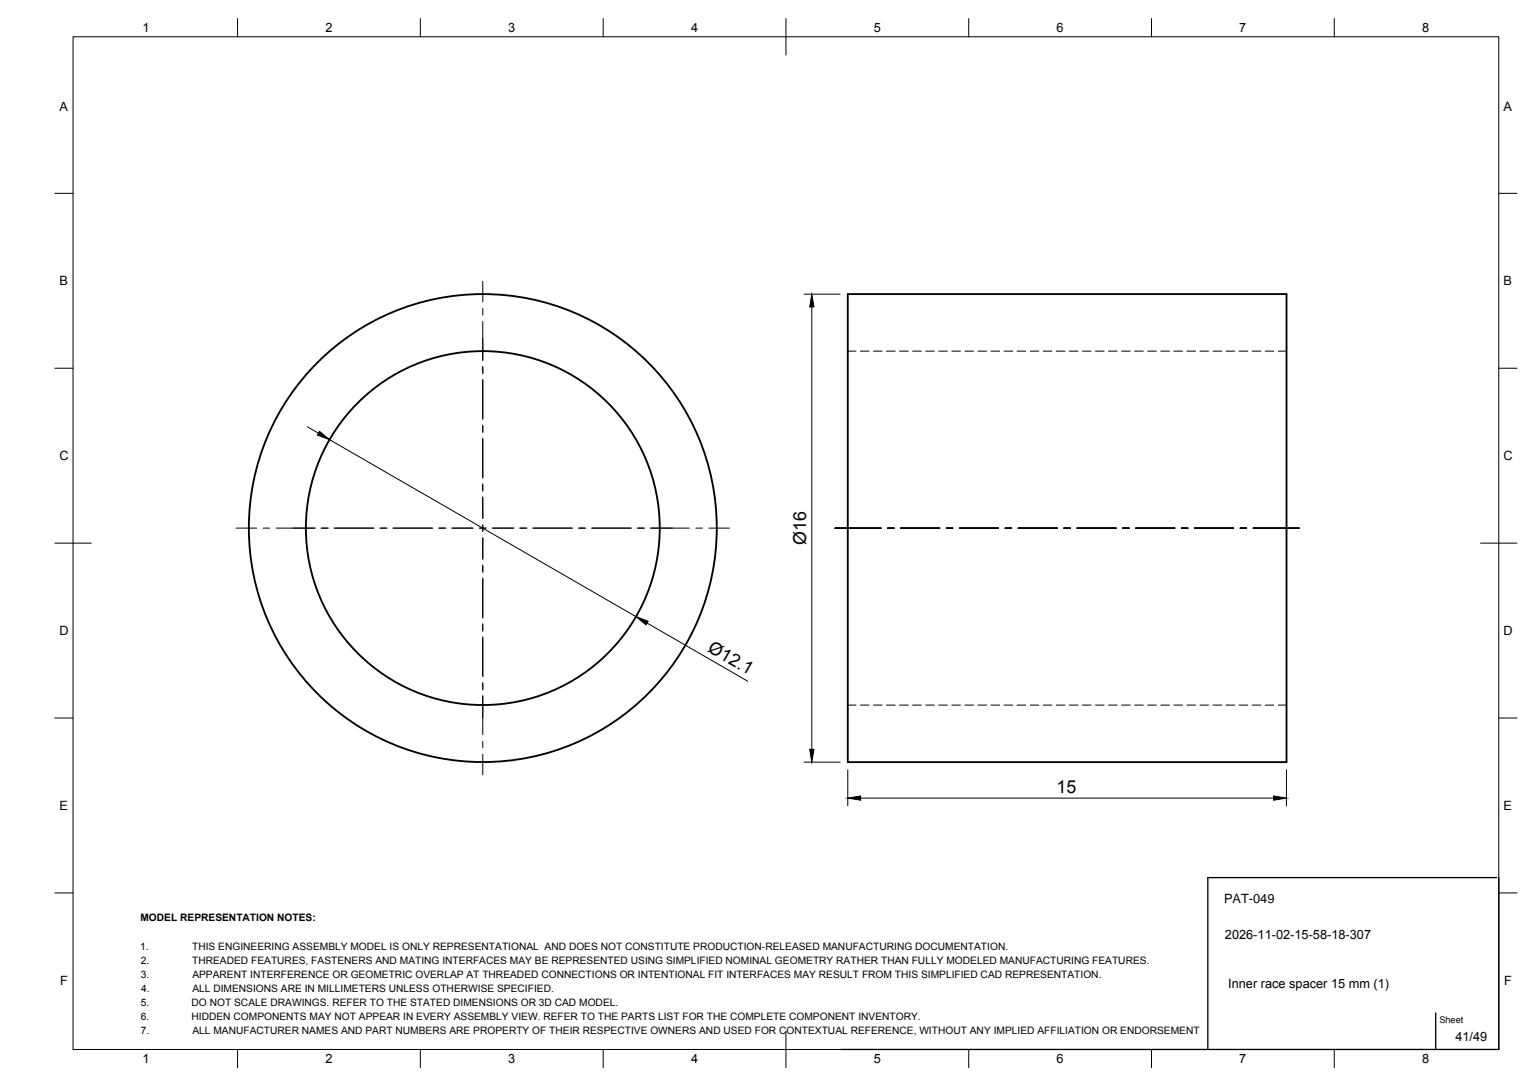
ISO-10303-21;
HEADER;
/* Generated by software containing ST-Developer
 * from STEP Tools, Inc. (www.steptools.com) 
 */

FILE_DESCRIPTION(
/* description */ ('Hand drill press frame (manual)'),
/* implementation_level */ '2;1');

FILE_NAME(
/* name */ 'Inner race spacer 15 mm (1).step',
/* time_stamp */ '2026-10-28T03:25:28-07:00',
/* author */ (''),
/* organization */ (''),
/* preprocessor_version */ 'ST-DEVELOPER v20.2',
/* originating_system */ 'Autodesk Translation Framework v15.17.0.0',
/* authorisation */ '');

FILE_SCHEMA (('AUTOMOTIVE_DESIGN { 1 0 10303 214 3 1 1 }'));
ENDSEC;

DATA;
#10=MECHANICAL_DESIGN_GEOMETRIC_PRESENTATION_REPRESENTATION('',(#659),#33299);
#562=SHAPE_REPRESENTATION_RELATIONSHIP('SRR','None',#33524,#607);
#607=ADVANCED_BREP_SHAPE_REPRESENTATION('',(#710),#33286);
#659=STYLED_ITEM('',(#33814),#710);
#710=MANIFOLD_SOLID_BREP('Body1',#12678);
#865=FACE_BOUND('',#2694,.T.);
#866=FACE_BOUND('',#2696,.T.);
#1258=PLANE('',#14067);
#1259=PLANE('',#14068);
#1857=FACE_OUTER_BOUND('',#2691,.T.);
#1858=FACE_OUTER_BOUND('',#2692,.T.);
#1859=FACE_OUTER_BOUND('',#2693,.T.);
#1860=FACE_OUTER_BOUND('',#2695,.T.);
#2691=EDGE_LOOP('',(#10967,#10968,#10969,#10970));
#2692=EDGE_LOOP('',(#10971,#10972,#10973,#10974));
#2693=EDGE_LOOP('',(#10975));
#2694=EDGE_LOOP('',(#10976));
#2695=EDGE_LOOP('',(#10977));
#2696=EDGE_LOOP('',(#10978));
#3814=LINE('',#21189,#4979);
#3815=LINE('',#21195,#4980);
#4979=VECTOR('',#17047,0.605);
#4980=VECTOR('',#17054,0.8);
#5519=CIRCLE('',#14062,0.605);
#5520=CIRCLE('',#14063,0.605);
#5521=CIRCLE('',#14065,0.8);
#5522=CIRCLE('',#14066,0.8);
#6469=VERTEX_POINT('',#21186);
#6470=VERTEX_POINT('',#21188);
#6471=VERTEX_POINT('',#21192);
#6472=VERTEX_POINT('',#21194);
#8012=EDGE_CURVE('',#6469,#6469,#5519,.T.);
#8013=EDGE_CURVE('',#6469,#6470,#3814,.T.);
#8014=EDGE_CURVE('',#6470,#6470,#5520,.T.);
#8015=EDGE_CURVE('',#6471,#6471,#5521,.T.);
#8016=EDGE_CURVE('',#6471,#6472,#3815,.T.);
#8017=EDGE_CURVE('',#6472,#6472,#5522,.T.);
#10967=ORIENTED_EDGE('',*,*,#8012,.F.);
#10968=ORIENTED_EDGE('',*,*,#8013,.T.);
#10969=ORIENTED_EDGE('',*,*,#8014,.T.);
#10970=ORIENTED_EDGE('',*,*,#8013,.F.);
#10971=ORIENTED_EDGE('',*,*,#8015,.F.);
#10972=ORIENTED_EDGE('',*,*,#8016,.T.);
#10973=ORIENTED_EDGE('',*,*,#8017,.T.);
#10974=ORIENTED_EDGE('',*,*,#8016,.F.);
#10975=ORIENTED_EDGE('',*,*,#8015,.T.);
#10976=ORIENTED_EDGE('',*,*,#8012,.T.);
#10977=ORIENTED_EDGE('',*,*,#8017,.F.);
#10978=ORIENTED_EDGE('',*,*,#8014,.F.);
#11906=CYLINDRICAL_SURFACE('',#14061,0.605);
#11907=CYLINDRICAL_SURFACE('',#14064,0.8);
#12466=ADVANCED_FACE('',(#1857),#11906,.F.);
#12467=ADVANCED_FACE('',(#1858),#11907,.T.);
#12468=ADVANCED_FACE('',(#1859,#865),#1258,.T.);
#12469=ADVANCED_FACE('',(#1860,#866),#1259,.F.);
#12678=CLOSED_SHELL('',(#12466,#12467,#12468,#12469));
#14060=AXIS2_PLACEMENT_3D('',#21184,#17041,#17042);
#14061=AXIS2_PLACEMENT_3D('',#21185,#17043,#17044);
#14062=AXIS2_PLACEMENT_3D('',#21187,#17045,#17046);
#14063=AXIS2_PLACEMENT_3D('',#21190,#17048,#17049);
#14064=AXIS2_PLACEMENT_3D('',#21191,#17050,#17051);
#14065=AXIS2_PLACEMENT_3D('',#21193,#17052,#17053);
#14066=AXIS2_PLACEMENT_3D('',#21196,#17055,#17056);
#14067=AXIS2_PLACEMENT_3D('',#21197,#17057,#17058);
#14068=AXIS2_PLACEMENT_3D('',#21198,#17059,#17060);
#17041=DIRECTION('axis',(0.,0.,1.));
#17042=DIRECTION('refdir',(1.,0.,0.));
#17043=DIRECTION('center_axis',(0.,1.,0.));
#17044=DIRECTION('ref_axis',(1.,0.,0.));
#17045=DIRECTION('center_axis',(0.,-1.,0.));
#17046=DIRECTION('ref_axis',(1.,0.,0.));
#17047=DIRECTION('',(0.,-1.,0.));
#17048=DIRECTION('center_axis',(0.,-1.,0.));
#17049=DIRECTION('ref_axis',(1.,0.,0.));
#17050=DIRECTION('center_axis',(0.,1.,0.));
#17051=DIRECTION('ref_axis',(1.,0.,0.));
#17052=DIRECTION('center_axis',(0.,1.,0.));
#17053=DIRECTION('ref_axis',(1.,0.,0.));
#17054=DIRECTION('',(0.,-1.,0.));
#17055=DIRECTION('center_axis',(0.,1.,0.));
#17056=DIRECTION('ref_axis',(1.,0.,0.));
#17057=DIRECTION('center_axis',(0.,1.,0.));
#17058=DIRECTION('ref_axis',(1.,0.,0.));
#17059=DIRECTION('center_axis',(0.,1.,0.));
#17060=DIRECTION('ref_axis',(1.,0.,0.));
#21184=CARTESIAN_POINT('',(0.,0.,0.));
#21185=CARTESIAN_POINT('Origin',(-3.25,3.5,20.));
#21186=CARTESIAN_POINT('',(-3.855,5.,20.));
#21187=CARTESIAN_POINT('Origin',(-3.25,5.,20.));
#21188=CARTESIAN_POINT('',(-3.855,3.5,20.));
#21189=CARTESIAN_POINT('',(-3.855,3.5,20.));
#21190=CARTESIAN_POINT('Origin',(-3.25,3.5,20.));
#21191=CARTESIAN_POINT('Origin',(-3.25,3.5,20.));
#21192=CARTESIAN_POINT('',(-4.05,5.,20.));
#21193=CARTESIAN_POINT('Origin',(-3.25,5.,20.));
#21194=CARTESIAN_POINT('',(-4.05,3.5,20.));
#21195=CARTESIAN_POINT('',(-4.05,3.5,20.));
#21196=CARTESIAN_POINT('Origin',(-3.25,3.5,20.));
#21197=CARTESIAN_POINT('Origin',(-3.25,5.,20.));
#21198=CARTESIAN_POINT('Origin',(-3.25,3.5,20.));
#33234=UNCERTAINTY_MEASURE_WITH_UNIT(LENGTH_MEASURE(0.001),#33300,
'DISTANCE_ACCURACY_VALUE',
'Maximum model space distance between geometric entities at asserted c
onnectivities');
#33247=UNCERTAINTY_MEASURE_WITH_UNIT(LENGTH_MEASURE(0.001),#33300,
'DISTANCE_ACCURACY_VALUE',
'Maximum model space distance between geometric entities at asserted c
onnectivities');
#33286=(
GEOMETRIC_REPRESENTATION_CONTEXT(3)
GLOBAL_UNCERTAINTY_ASSIGNED_CONTEXT((#33234))
GLOBAL_UNIT_ASSIGNED_CONTEXT((#33300,#33302,#33303))
REPRESENTATION_CONTEXT('','3D')
);
#33299=(
GEOMETRIC_REPRESENTATION_CONTEXT(3)
GLOBAL_UNCERTAINTY_ASSIGNED_CONTEXT((#33247))
GLOBAL_UNIT_ASSIGNED_CONTEXT((#33300,#33302,#33303))
REPRESENTATION_CONTEXT('','3D')
);
#33300=(
LENGTH_UNIT()
NAMED_UNIT(*)
SI_UNIT(.CENTI.,.METRE.)
);
#33302=(
NAMED_UNIT(*)
PLANE_ANGLE_UNIT()
SI_UNIT($,.RADIAN.)
);
#33303=(
NAMED_UNIT(*)
SI_UNIT($,.STERADIAN.)
SOLID_ANGLE_UNIT()
);
#33342=SHAPE_DEFINITION_REPRESENTATION(#33404,#33524);
#33404=PRODUCT_DEFINITION_SHAPE('',$,#33576);
#33524=SHAPE_REPRESENTATION('',(#14060),#33286);
#33537=PRODUCT_DEFINITION_CONTEXT('part definition',#33692,'design');
#33576=PRODUCT_DEFINITION('Inner race spacer 15 mm (1)',
'Inner race spacer 15 mm (1)',#33627,#33537);
#33627=PRODUCT_DEFINITION_FORMATION('',$,#33732);
#33692=APPLICATION_CONTEXT(
'Core Data for Automotive Mechanical Design Process');
#33693=PRODUCT_CONTEXT('part definition',#33692,'mechanical');
#33732=PRODUCT('Inner race spacer 15 mm (1)',
'Inner race spacer 15 mm (1)','Inner race spacer 15 mm (1)',(#33693));
#33808=COLOUR_RGB('Grey',0.48,0.52,0.57);
#33809=FILL_AREA_STYLE_COLOUR('',#33808);
#33810=FILL_AREA_STYLE('',(#33809));
#33811=SURFACE_STYLE_FILL_AREA(#33810);
#33812=SURFACE_SIDE_STYLE('',(#33811));
#33813=SURFACE_STYLE_USAGE(.BOTH.,#33812);
#33814=PRESENTATION_STYLE_ASSIGNMENT((#33813));
ENDSEC;
END-ISO-10303-21;
